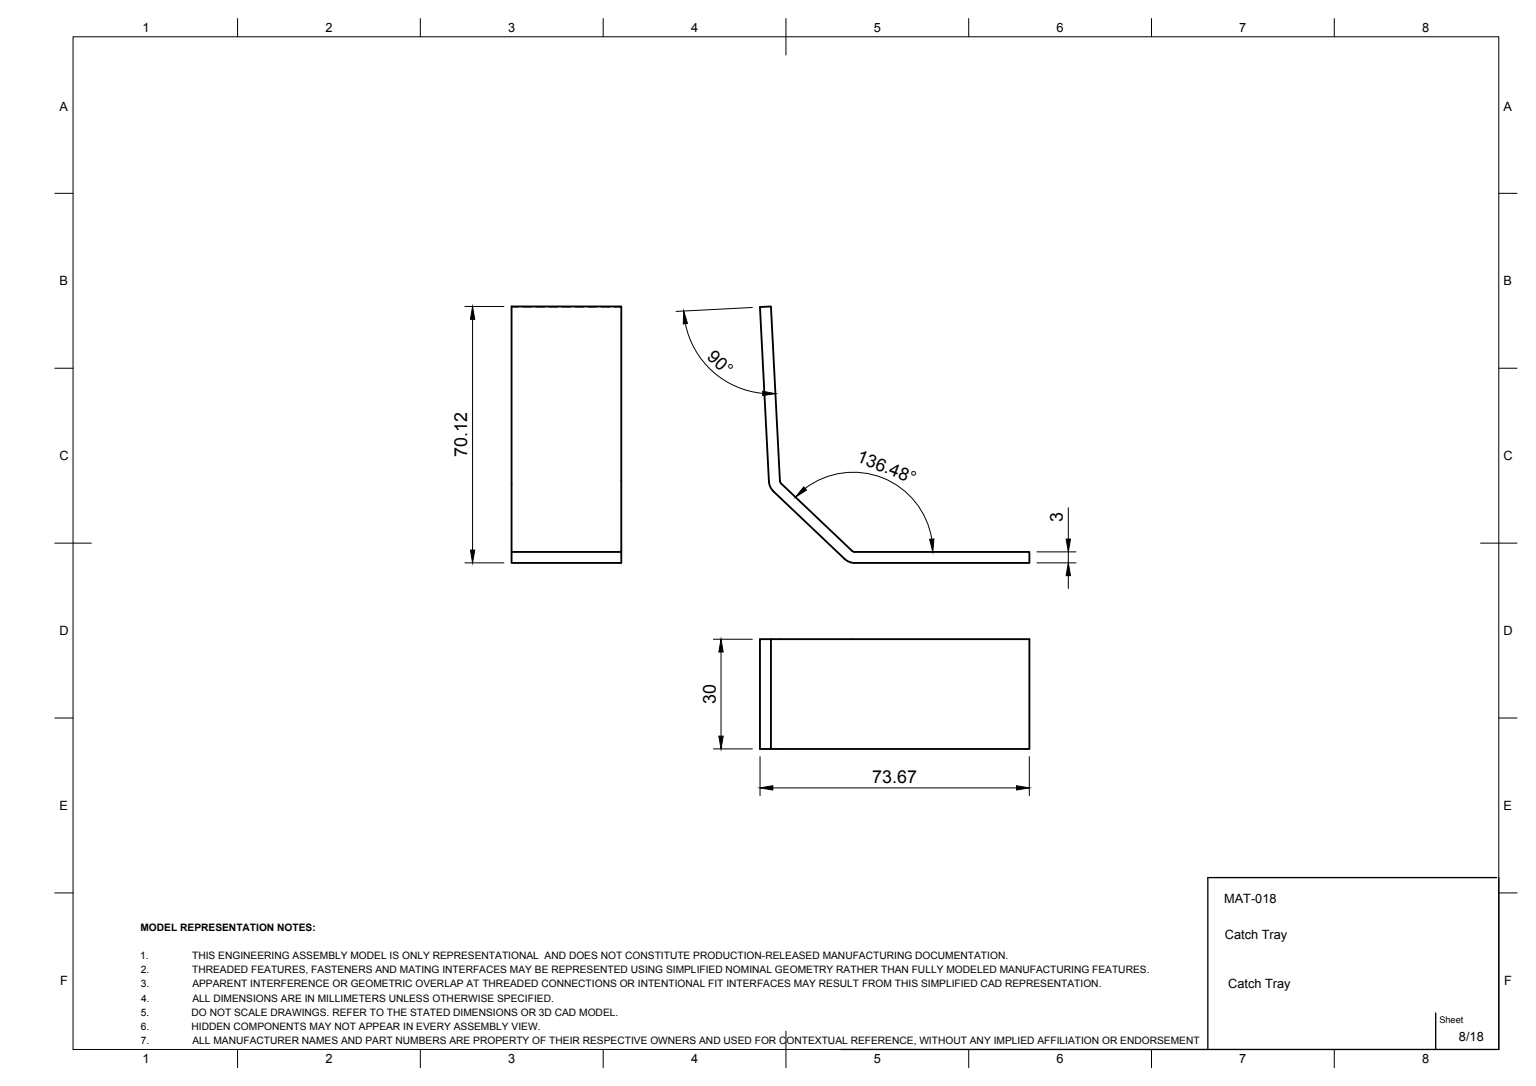
ISO-10303-21;
HEADER;
/* Generated by software containing ST-Developer
 * from STEP Tools, Inc. (www.steptools.com) 
 */

FILE_DESCRIPTION(
/* description */ ('STEP AP214'),
/* implementation_level */ '2;1');

FILE_NAME(
/* name */ 'Catch Tray.step',
/* time_stamp */ '2026-11-14T06:16:09-08:00',
/* author */ (''),
/* organization */ (''),
/* preprocessor_version */ 'ST-DEVELOPER v20.2',
/* originating_system */ 'Autodesk Translation Framework v15.17.0.0',
/* authorisation */ '');

FILE_SCHEMA (('AUTOMOTIVE_DESIGN { 1 0 10303 214 3 1 1 }'));
ENDSEC;

DATA;
#10=MECHANICAL_DESIGN_GEOMETRIC_PRESENTATION_REPRESENTATION('',(#352),#18006);
#320=SHAPE_REPRESENTATION_RELATIONSHIP('SRR','None',#18076,#336);
#336=ADVANCED_BREP_SHAPE_REPRESENTATION('',(#368),#17993);
#352=STYLED_ITEM('',(#18170),#368);
#368=MANIFOLD_SOLID_BREP('Body1',#9561);
#692=PLANE('',#10212);
#693=PLANE('',#10215);
#694=PLANE('',#10216);
#695=PLANE('',#10219);
#696=PLANE('',#10220);
#697=PLANE('',#10223);
#698=PLANE('',#10224);
#699=PLANE('',#10227);
#700=PLANE('',#10228);
#701=PLANE('',#10229);
#702=PLANE('',#10230);
#703=PLANE('',#10232);
#704=PLANE('',#10234);
#705=PLANE('',#10235);
#706=PLANE('',#10236);
#707=PLANE('',#10238);
#708=PLANE('',#10240);
#709=PLANE('',#10241);
#1117=FACE_OUTER_BOUND('',#1769,.T.);
#1118=FACE_OUTER_BOUND('',#1770,.T.);
#1119=FACE_OUTER_BOUND('',#1771,.T.);
#1120=FACE_OUTER_BOUND('',#1772,.T.);
#1121=FACE_OUTER_BOUND('',#1773,.T.);
#1122=FACE_OUTER_BOUND('',#1774,.T.);
#1123=FACE_OUTER_BOUND('',#1775,.T.);
#1124=FACE_OUTER_BOUND('',#1776,.T.);
#1125=FACE_OUTER_BOUND('',#1777,.T.);
#1126=FACE_OUTER_BOUND('',#1778,.T.);
#1127=FACE_OUTER_BOUND('',#1779,.T.);
#1128=FACE_OUTER_BOUND('',#1780,.T.);
#1129=FACE_OUTER_BOUND('',#1781,.T.);
#1130=FACE_OUTER_BOUND('',#1782,.T.);
#1131=FACE_OUTER_BOUND('',#1783,.T.);
#1132=FACE_OUTER_BOUND('',#1784,.T.);
#1133=FACE_OUTER_BOUND('',#1785,.T.);
#1134=FACE_OUTER_BOUND('',#1786,.T.);
#1135=FACE_OUTER_BOUND('',#1787,.T.);
#1136=FACE_OUTER_BOUND('',#1788,.T.);
#1137=FACE_OUTER_BOUND('',#1789,.T.);
#1138=FACE_OUTER_BOUND('',#1790,.T.);
#1769=EDGE_LOOP('',(#7428,#7429,#7430,#7431));
#1770=EDGE_LOOP('',(#7432,#7433,#7434,#7435));
#1771=EDGE_LOOP('',(#7436,#7437,#7438,#7439));
#1772=EDGE_LOOP('',(#7440,#7441,#7442,#7443));
#1773=EDGE_LOOP('',(#7444,#7445,#7446,#7447));
#1774=EDGE_LOOP('',(#7448,#7449,#7450,#7451));
#1775=EDGE_LOOP('',(#7452,#7453,#7454,#7455));
#1776=EDGE_LOOP('',(#7456,#7457,#7458,#7459));
#1777=EDGE_LOOP('',(#7460,#7461,#7462,#7463));
#1778=EDGE_LOOP('',(#7464,#7465,#7466,#7467));
#1779=EDGE_LOOP('',(#7468,#7469,#7470,#7471));
#1780=EDGE_LOOP('',(#7472,#7473,#7474,#7475));
#1781=EDGE_LOOP('',(#7476,#7477,#7478,#7479));
#1782=EDGE_LOOP('',(#7480,#7481,#7482,#7483));
#1783=EDGE_LOOP('',(#7484,#7485,#7486,#7487));
#1784=EDGE_LOOP('',(#7488,#7489,#7490,#7491));
#1785=EDGE_LOOP('',(#7492,#7493,#7494,#7495));
#1786=EDGE_LOOP('',(#7496,#7497,#7498,#7499));
#1787=EDGE_LOOP('',(#7500,#7501,#7502,#7503));
#1788=EDGE_LOOP('',(#7504,#7505,#7506,#7507));
#1789=EDGE_LOOP('',(#7508,#7509,#7510,#7511));
#1790=EDGE_LOOP('',(#7512,#7513,#7514,#7515));
#2574=LINE('',#15105,#3298);
#2575=LINE('',#15109,#3299);
#2576=LINE('',#15113,#3300);
#2577=LINE('',#15115,#3301);
#2578=LINE('',#15116,#3302);
#2579=LINE('',#15120,#3303);
#2580=LINE('',#15124,#3304);
#2581=LINE('',#15128,#3305);
#2582=LINE('',#15130,#3306);
#2583=LINE('',#15131,#3307);
#2584=LINE('',#15135,#3308);
#2585=LINE('',#15140,#3309);
#2586=LINE('',#15142,#3310);
#2587=LINE('',#15143,#3311);
#2588=LINE('',#15147,#3312);
#2589=LINE('',#15151,#3313);
#2590=LINE('',#15154,#3314);
#2591=LINE('',#15155,#3315);
#2592=LINE('',#15158,#3316);
#2593=LINE('',#15159,#3317);
#2594=LINE('',#15160,#3318);
#2595=LINE('',#15163,#3319);
#2596=LINE('',#15164,#3320);
#2597=LINE('',#15166,#3321);
#2598=LINE('',#15167,#3322);
#2599=LINE('',#15169,#3323);
#2600=LINE('',#15171,#3324);
#2601=LINE('',#15173,#3325);
#2602=LINE('',#15176,#3326);
#2603=LINE('',#15177,#3327);
#2604=LINE('',#15180,#3328);
#2605=LINE('',#15181,#3329);
#2606=LINE('',#15183,#3330);
#2607=LINE('',#15184,#3331);
#2608=LINE('',#15186,#3332);
#2609=LINE('',#15188,#3333);
#3298=VECTOR('',#12247,1000.);
#3299=VECTOR('',#12250,1000.);
#3300=VECTOR('',#12255,1000.);
#3301=VECTOR('',#12256,1000.);
#3302=VECTOR('',#12257,1000.);
#3303=VECTOR('',#12260,1000.);
#3304=VECTOR('',#12263,1000.);
#3305=VECTOR('',#12268,1000.);
#3306=VECTOR('',#12269,1000.);
#3307=VECTOR('',#12270,1000.);
#3308=VECTOR('',#12273,1000.);
#3309=VECTOR('',#12280,1000.);
#3310=VECTOR('',#12281,1000.);
#3311=VECTOR('',#12282,1000.);
#3312=VECTOR('',#12285,1000.);
#3313=VECTOR('',#12288,1000.);
#3314=VECTOR('',#12293,1000.);
#3315=VECTOR('',#12294,1000.);
#3316=VECTOR('',#12297,1000.);
#3317=VECTOR('',#12298,1000.);
#3318=VECTOR('',#12299,1000.);
#3319=VECTOR('',#12302,1000.);
#3320=VECTOR('',#12303,1000.);
#3321=VECTOR('',#12306,1000.);
#3322=VECTOR('',#12307,1000.);
#3323=VECTOR('',#12310,1000.);
#3324=VECTOR('',#12313,1000.);
#3325=VECTOR('',#12316,1000.);
#3326=VECTOR('',#12319,1000.);
#3327=VECTOR('',#12320,1000.);
#3328=VECTOR('',#12323,1000.);
#3329=VECTOR('',#12324,1000.);
#3330=VECTOR('',#12327,1000.);
#3331=VECTOR('',#12328,1000.);
#3332=VECTOR('',#12331,1000.);
#3333=VECTOR('',#12334,1000.);
#3736=CIRCLE('',#10213,4.);
#3737=CIRCLE('',#10214,1.);
#3738=CIRCLE('',#10217,4.);
#3739=CIRCLE('',#10218,1.);
#3740=CIRCLE('',#10221,4.);
#3741=CIRCLE('',#10222,1.);
#3742=CIRCLE('',#10225,4.);
#3743=CIRCLE('',#10226,1.);
#4385=VERTEX_POINT('',#15103);
#4386=VERTEX_POINT('',#15104);
#4387=VERTEX_POINT('',#15106);
#4388=VERTEX_POINT('',#15108);
#4389=VERTEX_POINT('',#15112);
#4390=VERTEX_POINT('',#15114);
#4391=VERTEX_POINT('',#15118);
#4392=VERTEX_POINT('',#15119);
#4393=VERTEX_POINT('',#15121);
#4394=VERTEX_POINT('',#15123);
#4395=VERTEX_POINT('',#15127);
#4396=VERTEX_POINT('',#15129);
#4397=VERTEX_POINT('',#15133);
#4398=VERTEX_POINT('',#15134);
#4399=VERTEX_POINT('',#15139);
#4400=VERTEX_POINT('',#15141);
#4401=VERTEX_POINT('',#15145);
#4402=VERTEX_POINT('',#15146);
#4403=VERTEX_POINT('',#15148);
#4404=VERTEX_POINT('',#15150);
#4405=VERTEX_POINT('',#15157);
#4406=VERTEX_POINT('',#15162);
#4407=VERTEX_POINT('',#15175);
#4408=VERTEX_POINT('',#15179);
#5462=EDGE_CURVE('',#4385,#4386,#2574,.T.);
#5463=EDGE_CURVE('',#4387,#4385,#3736,.T.);
#5464=EDGE_CURVE('',#4388,#4387,#2575,.T.);
#5465=EDGE_CURVE('',#4388,#4386,#3737,.T.);
#5466=EDGE_CURVE('',#4385,#4389,#2576,.T.);
#5467=EDGE_CURVE('',#4386,#4390,#2577,.T.);
#5468=EDGE_CURVE('',#4390,#4389,#2578,.T.);
#5469=EDGE_CURVE('',#4391,#4392,#2579,.T.);
#5470=EDGE_CURVE('',#4391,#4393,#3738,.T.);
#5471=EDGE_CURVE('',#4394,#4393,#2580,.T.);
#5472=EDGE_CURVE('',#4392,#4394,#3739,.T.);
#5473=EDGE_CURVE('',#4395,#4391,#2581,.T.);
#5474=EDGE_CURVE('',#4396,#4392,#2582,.T.);
#5475=EDGE_CURVE('',#4396,#4395,#2583,.T.);
#5476=EDGE_CURVE('',#4397,#4398,#2584,.T.);
#5477=EDGE_CURVE('',#4389,#4397,#3740,.T.);
#5478=EDGE_CURVE('',#4390,#4398,#3741,.T.);
#5479=EDGE_CURVE('',#4397,#4399,#2585,.T.);
#5480=EDGE_CURVE('',#4398,#4400,#2586,.T.);
#5481=EDGE_CURVE('',#4399,#4400,#2587,.T.);
#5482=EDGE_CURVE('',#4401,#4402,#2588,.T.);
#5483=EDGE_CURVE('',#4401,#4403,#3742,.T.);
#5484=EDGE_CURVE('',#4404,#4403,#2589,.T.);
#5485=EDGE_CURVE('',#4402,#4404,#3743,.T.);
#5486=EDGE_CURVE('',#4393,#4401,#2590,.T.);
#5487=EDGE_CURVE('',#4394,#4402,#2591,.T.);
#5488=EDGE_CURVE('',#4404,#4405,#2592,.T.);
#5489=EDGE_CURVE('',#4400,#4405,#2593,.T.);
#5490=EDGE_CURVE('',#4398,#4404,#2594,.T.);
#5491=EDGE_CURVE('',#4406,#4405,#2595,.T.);
#5492=EDGE_CURVE('',#4399,#4406,#2596,.T.);
#5493=EDGE_CURVE('',#4403,#4406,#2597,.T.);
#5494=EDGE_CURVE('',#4397,#4403,#2598,.T.);
#5495=EDGE_CURVE('',#4389,#4401,#2599,.T.);
#5496=EDGE_CURVE('',#4385,#4393,#2600,.T.);
#5497=EDGE_CURVE('',#4387,#4391,#2601,.T.);
#5498=EDGE_CURVE('',#4407,#4395,#2602,.T.);
#5499=EDGE_CURVE('',#4407,#4387,#2603,.T.);
#5500=EDGE_CURVE('',#4408,#4396,#2604,.T.);
#5501=EDGE_CURVE('',#4408,#4407,#2605,.T.);
#5502=EDGE_CURVE('',#4388,#4392,#2606,.T.);
#5503=EDGE_CURVE('',#4408,#4388,#2607,.T.);
#5504=EDGE_CURVE('',#4386,#4394,#2608,.T.);
#5505=EDGE_CURVE('',#4390,#4402,#2609,.T.);
#7428=ORIENTED_EDGE('',*,*,#5462,.F.);
#7429=ORIENTED_EDGE('',*,*,#5463,.F.);
#7430=ORIENTED_EDGE('',*,*,#5464,.F.);
#7431=ORIENTED_EDGE('',*,*,#5465,.T.);
#7432=ORIENTED_EDGE('',*,*,#5466,.F.);
#7433=ORIENTED_EDGE('',*,*,#5462,.T.);
#7434=ORIENTED_EDGE('',*,*,#5467,.T.);
#7435=ORIENTED_EDGE('',*,*,#5468,.T.);
#7436=ORIENTED_EDGE('',*,*,#5469,.F.);
#7437=ORIENTED_EDGE('',*,*,#5470,.T.);
#7438=ORIENTED_EDGE('',*,*,#5471,.F.);
#7439=ORIENTED_EDGE('',*,*,#5472,.F.);
#7440=ORIENTED_EDGE('',*,*,#5473,.T.);
#7441=ORIENTED_EDGE('',*,*,#5469,.T.);
#7442=ORIENTED_EDGE('',*,*,#5474,.F.);
#7443=ORIENTED_EDGE('',*,*,#5475,.T.);
#7444=ORIENTED_EDGE('',*,*,#5476,.F.);
#7445=ORIENTED_EDGE('',*,*,#5477,.F.);
#7446=ORIENTED_EDGE('',*,*,#5468,.F.);
#7447=ORIENTED_EDGE('',*,*,#5478,.T.);
#7448=ORIENTED_EDGE('',*,*,#5479,.F.);
#7449=ORIENTED_EDGE('',*,*,#5476,.T.);
#7450=ORIENTED_EDGE('',*,*,#5480,.T.);
#7451=ORIENTED_EDGE('',*,*,#5481,.F.);
#7452=ORIENTED_EDGE('',*,*,#5482,.F.);
#7453=ORIENTED_EDGE('',*,*,#5483,.T.);
#7454=ORIENTED_EDGE('',*,*,#5484,.F.);
#7455=ORIENTED_EDGE('',*,*,#5485,.F.);
#7456=ORIENTED_EDGE('',*,*,#5486,.T.);
#7457=ORIENTED_EDGE('',*,*,#5482,.T.);
#7458=ORIENTED_EDGE('',*,*,#5487,.F.);
#7459=ORIENTED_EDGE('',*,*,#5471,.T.);
#7460=ORIENTED_EDGE('',*,*,#5488,.T.);
#7461=ORIENTED_EDGE('',*,*,#5489,.F.);
#7462=ORIENTED_EDGE('',*,*,#5480,.F.);
#7463=ORIENTED_EDGE('',*,*,#5490,.T.);
#7464=ORIENTED_EDGE('',*,*,#5491,.F.);
#7465=ORIENTED_EDGE('',*,*,#5492,.F.);
#7466=ORIENTED_EDGE('',*,*,#5481,.T.);
#7467=ORIENTED_EDGE('',*,*,#5489,.T.);
#7468=ORIENTED_EDGE('',*,*,#5493,.F.);
#7469=ORIENTED_EDGE('',*,*,#5494,.F.);
#7470=ORIENTED_EDGE('',*,*,#5479,.T.);
#7471=ORIENTED_EDGE('',*,*,#5492,.T.);
#7472=ORIENTED_EDGE('',*,*,#5483,.F.);
#7473=ORIENTED_EDGE('',*,*,#5495,.F.);
#7474=ORIENTED_EDGE('',*,*,#5477,.T.);
#7475=ORIENTED_EDGE('',*,*,#5494,.T.);
#7476=ORIENTED_EDGE('',*,*,#5486,.F.);
#7477=ORIENTED_EDGE('',*,*,#5496,.F.);
#7478=ORIENTED_EDGE('',*,*,#5466,.T.);
#7479=ORIENTED_EDGE('',*,*,#5495,.T.);
#7480=ORIENTED_EDGE('',*,*,#5470,.F.);
#7481=ORIENTED_EDGE('',*,*,#5497,.F.);
#7482=ORIENTED_EDGE('',*,*,#5463,.T.);
#7483=ORIENTED_EDGE('',*,*,#5496,.T.);
#7484=ORIENTED_EDGE('',*,*,#5473,.F.);
#7485=ORIENTED_EDGE('',*,*,#5498,.F.);
#7486=ORIENTED_EDGE('',*,*,#5499,.T.);
#7487=ORIENTED_EDGE('',*,*,#5497,.T.);
#7488=ORIENTED_EDGE('',*,*,#5475,.F.);
#7489=ORIENTED_EDGE('',*,*,#5500,.F.);
#7490=ORIENTED_EDGE('',*,*,#5501,.T.);
#7491=ORIENTED_EDGE('',*,*,#5498,.T.);
#7492=ORIENTED_EDGE('',*,*,#5474,.T.);
#7493=ORIENTED_EDGE('',*,*,#5502,.F.);
#7494=ORIENTED_EDGE('',*,*,#5503,.F.);
#7495=ORIENTED_EDGE('',*,*,#5500,.T.);
#7496=ORIENTED_EDGE('',*,*,#5472,.T.);
#7497=ORIENTED_EDGE('',*,*,#5504,.F.);
#7498=ORIENTED_EDGE('',*,*,#5465,.F.);
#7499=ORIENTED_EDGE('',*,*,#5502,.T.);
#7500=ORIENTED_EDGE('',*,*,#5487,.T.);
#7501=ORIENTED_EDGE('',*,*,#5505,.F.);
#7502=ORIENTED_EDGE('',*,*,#5467,.F.);
#7503=ORIENTED_EDGE('',*,*,#5504,.T.);
#7504=ORIENTED_EDGE('',*,*,#5485,.T.);
#7505=ORIENTED_EDGE('',*,*,#5490,.F.);
#7506=ORIENTED_EDGE('',*,*,#5478,.F.);
#7507=ORIENTED_EDGE('',*,*,#5505,.T.);
#7508=ORIENTED_EDGE('',*,*,#5503,.T.);
#7509=ORIENTED_EDGE('',*,*,#5464,.T.);
#7510=ORIENTED_EDGE('',*,*,#5499,.F.);
#7511=ORIENTED_EDGE('',*,*,#5501,.F.);
#7512=ORIENTED_EDGE('',*,*,#5488,.F.);
#7513=ORIENTED_EDGE('',*,*,#5484,.T.);
#7514=ORIENTED_EDGE('',*,*,#5493,.T.);
#7515=ORIENTED_EDGE('',*,*,#5491,.T.);
#8894=CYLINDRICAL_SURFACE('',#10231,4.);
#8895=CYLINDRICAL_SURFACE('',#10233,4.);
#8896=CYLINDRICAL_SURFACE('',#10237,1.);
#8897=CYLINDRICAL_SURFACE('',#10239,1.);
#9256=ADVANCED_FACE('',(#1117),#692,.T.);
#9257=ADVANCED_FACE('',(#1118),#693,.T.);
#9258=ADVANCED_FACE('',(#1119),#694,.T.);
#9259=ADVANCED_FACE('',(#1120),#695,.T.);
#9260=ADVANCED_FACE('',(#1121),#696,.T.);
#9261=ADVANCED_FACE('',(#1122),#697,.T.);
#9262=ADVANCED_FACE('',(#1123),#698,.T.);
#9263=ADVANCED_FACE('',(#1124),#699,.T.);
#9264=ADVANCED_FACE('',(#1125),#700,.F.);
#9265=ADVANCED_FACE('',(#1126),#701,.T.);
#9266=ADVANCED_FACE('',(#1127),#702,.T.);
#9267=ADVANCED_FACE('',(#1128),#8894,.T.);
#9268=ADVANCED_FACE('',(#1129),#703,.T.);
#9269=ADVANCED_FACE('',(#1130),#8895,.T.);
#9270=ADVANCED_FACE('',(#1131),#704,.T.);
#9271=ADVANCED_FACE('',(#1132),#705,.T.);
#9272=ADVANCED_FACE('',(#1133),#706,.F.);
#9273=ADVANCED_FACE('',(#1134),#8896,.F.);
#9274=ADVANCED_FACE('',(#1135),#707,.F.);
#9275=ADVANCED_FACE('',(#1136),#8897,.F.);
#9276=ADVANCED_FACE('',(#1137),#708,.T.);
#9277=ADVANCED_FACE('',(#1138),#709,.F.);
#9561=CLOSED_SHELL('',(#9256,#9257,#9258,#9259,#9260,#9261,#9262,#9263,
#9264,#9265,#9266,#9267,#9268,#9269,#9270,#9271,#9272,#9273,#9274,#9275,
#9276,#9277));
#10211=AXIS2_PLACEMENT_3D('',#15101,#12243,#12244);
#10212=AXIS2_PLACEMENT_3D('',#15102,#12245,#12246);
#10213=AXIS2_PLACEMENT_3D('',#15107,#12248,#12249);
#10214=AXIS2_PLACEMENT_3D('',#15110,#12251,#12252);
#10215=AXIS2_PLACEMENT_3D('',#15111,#12253,#12254);
#10216=AXIS2_PLACEMENT_3D('',#15117,#12258,#12259);
#10217=AXIS2_PLACEMENT_3D('',#15122,#12261,#12262);
#10218=AXIS2_PLACEMENT_3D('',#15125,#12264,#12265);
#10219=AXIS2_PLACEMENT_3D('',#15126,#12266,#12267);
#10220=AXIS2_PLACEMENT_3D('',#15132,#12271,#12272);
#10221=AXIS2_PLACEMENT_3D('',#15136,#12274,#12275);
#10222=AXIS2_PLACEMENT_3D('',#15137,#12276,#12277);
#10223=AXIS2_PLACEMENT_3D('',#15138,#12278,#12279);
#10224=AXIS2_PLACEMENT_3D('',#15144,#12283,#12284);
#10225=AXIS2_PLACEMENT_3D('',#15149,#12286,#12287);
#10226=AXIS2_PLACEMENT_3D('',#15152,#12289,#12290);
#10227=AXIS2_PLACEMENT_3D('',#15153,#12291,#12292);
#10228=AXIS2_PLACEMENT_3D('',#15156,#12295,#12296);
#10229=AXIS2_PLACEMENT_3D('',#15161,#12300,#12301);
#10230=AXIS2_PLACEMENT_3D('',#15165,#12304,#12305);
#10231=AXIS2_PLACEMENT_3D('',#15168,#12308,#12309);
#10232=AXIS2_PLACEMENT_3D('',#15170,#12311,#12312);
#10233=AXIS2_PLACEMENT_3D('',#15172,#12314,#12315);
#10234=AXIS2_PLACEMENT_3D('',#15174,#12317,#12318);
#10235=AXIS2_PLACEMENT_3D('',#15178,#12321,#12322);
#10236=AXIS2_PLACEMENT_3D('',#15182,#12325,#12326);
#10237=AXIS2_PLACEMENT_3D('',#15185,#12329,#12330);
#10238=AXIS2_PLACEMENT_3D('',#15187,#12332,#12333);
#10239=AXIS2_PLACEMENT_3D('',#15189,#12335,#12336);
#10240=AXIS2_PLACEMENT_3D('',#15190,#12337,#12338);
#10241=AXIS2_PLACEMENT_3D('',#15191,#12339,#12340);
#12243=DIRECTION('axis',(0.,0.,1.));
#12244=DIRECTION('refdir',(1.,0.,0.));
#12245=DIRECTION('center_axis',(0.,0.,1.));
#12246=DIRECTION('ref_axis',(1.,0.,0.));
#12247=DIRECTION('',(0.,-1.,0.));
#12248=DIRECTION('center_axis',(0.,0.,-1.));
#12249=DIRECTION('ref_axis',(1.,0.,0.));
#12250=DIRECTION('',(-0.688642993486688,0.72510056373009,0.));
#12251=DIRECTION('center_axis',(0.,0.,-1.));
#12252=DIRECTION('ref_axis',(1.,0.,0.));
#12253=DIRECTION('center_axis',(0.,0.,1.));
#12254=DIRECTION('ref_axis',(1.,0.,0.));
#12255=DIRECTION('',(1.,0.,0.));
#12256=DIRECTION('',(1.,0.,0.));
#12257=DIRECTION('',(0.,1.,0.));
#12258=DIRECTION('center_axis',(0.,0.,-1.));
#12259=DIRECTION('ref_axis',(-1.,0.,0.));
#12260=DIRECTION('',(0.688642993486688,-0.72510056373009,0.));
#12261=DIRECTION('center_axis',(0.,0.,-1.));
#12262=DIRECTION('ref_axis',(1.,0.,0.));
#12263=DIRECTION('',(0.,1.,0.));
#12264=DIRECTION('center_axis',(0.,0.,-1.));
#12265=DIRECTION('ref_axis',(1.,0.,0.));
#12266=DIRECTION('center_axis',(0.,0.,-1.));
#12267=DIRECTION('ref_axis',(-1.,0.,0.));
#12268=DIRECTION('',(0.725100563730095,0.688642993486682,0.));
#12269=DIRECTION('',(0.725100563730095,0.688642993486682,0.));
#12270=DIRECTION('',(-0.688642993486682,0.725100563730095,0.));
#12271=DIRECTION('center_axis',(0.,0.,1.));
#12272=DIRECTION('ref_axis',(1.,0.,0.));
#12273=DIRECTION('',(-0.688642993486681,-0.725100563730095,0.));
#12274=DIRECTION('center_axis',(0.,0.,-1.));
#12275=DIRECTION('ref_axis',(1.,-1.73472347597681E-15,0.));
#12276=DIRECTION('center_axis',(0.,0.,-1.));
#12277=DIRECTION('ref_axis',(1.,0.,0.));
#12278=DIRECTION('center_axis',(0.,0.,1.));
#12279=DIRECTION('ref_axis',(1.,0.,0.));
#12280=DIRECTION('',(0.725100563730095,-0.688642993486682,0.));
#12281=DIRECTION('',(0.725100563730095,-0.688642993486682,0.));
#12282=DIRECTION('',(-0.688642993486681,-0.725100563730095,0.));
#12283=DIRECTION('center_axis',(0.,0.,-1.));
#12284=DIRECTION('ref_axis',(-1.,0.,0.));
#12285=DIRECTION('',(0.,-1.,0.));
#12286=DIRECTION('center_axis',(0.,0.,-1.));
#12287=DIRECTION('ref_axis',(1.,-1.73472347597681E-15,0.));
#12288=DIRECTION('',(0.688642993486681,0.725100563730095,0.));
#12289=DIRECTION('center_axis',(0.,0.,-1.));
#12290=DIRECTION('ref_axis',(1.,0.,0.));
#12291=DIRECTION('center_axis',(0.,0.,-1.));
#12292=DIRECTION('ref_axis',(-1.,0.,0.));
#12293=DIRECTION('',(1.,0.,0.));
#12294=DIRECTION('',(1.,0.,0.));
#12295=DIRECTION('center_axis',(0.688642993486682,0.725100563730095,0.));
#12296=DIRECTION('ref_axis',(-0.725100563730095,0.688642993486682,0.));
#12297=DIRECTION('',(0.725100563730095,-0.688642993486682,0.));
#12298=DIRECTION('',(0.,0.,-1.));
#12299=DIRECTION('',(0.,0.,-1.));
#12300=DIRECTION('center_axis',(0.725100563730096,-0.688642993486682,0.));
#12301=DIRECTION('ref_axis',(0.688642993486682,0.725100563730096,0.));
#12302=DIRECTION('',(-0.688642993486681,-0.725100563730095,0.));
#12303=DIRECTION('',(0.,0.,-1.));
#12304=DIRECTION('center_axis',(0.688642993486682,0.725100563730095,0.));
#12305=DIRECTION('ref_axis',(-0.725100563730095,0.688642993486682,0.));
#12306=DIRECTION('',(0.725100563730095,-0.688642993486682,0.));
#12307=DIRECTION('',(0.,0.,-1.));
#12308=DIRECTION('center_axis',(0.,0.,-1.));
#12309=DIRECTION('ref_axis',(-1.,0.,0.));
#12310=DIRECTION('',(0.,0.,-1.));
#12311=DIRECTION('center_axis',(0.,1.,0.));
#12312=DIRECTION('ref_axis',(0.,0.,1.));
#12313=DIRECTION('',(0.,0.,-1.));
#12314=DIRECTION('center_axis',(0.,0.,-1.));
#12315=DIRECTION('ref_axis',(-1.,0.,0.));
#12316=DIRECTION('',(0.,0.,-1.));
#12317=DIRECTION('center_axis',(-0.688642993486682,0.725100563730095,0.));
#12318=DIRECTION('ref_axis',(-0.725100563730095,-0.688642993486682,0.));
#12319=DIRECTION('',(0.,0.,-1.));
#12320=DIRECTION('',(0.725100563730095,0.688642993486682,0.));
#12321=DIRECTION('center_axis',(-0.725100563730095,-0.688642993486682,0.));
#12322=DIRECTION('ref_axis',(0.688642993486682,-0.725100563730095,0.));
#12323=DIRECTION('',(0.,0.,-1.));
#12324=DIRECTION('',(-0.688642993486682,0.725100563730095,0.));
#12325=DIRECTION('center_axis',(-0.688642993486682,0.725100563730095,0.));
#12326=DIRECTION('ref_axis',(-0.725100563730095,-0.688642993486682,0.));
#12327=DIRECTION('',(0.,0.,-1.));
#12328=DIRECTION('',(0.725100563730095,0.688642993486682,0.));
#12329=DIRECTION('center_axis',(0.,0.,-1.));
#12330=DIRECTION('ref_axis',(-1.,0.,0.));
#12331=DIRECTION('',(0.,0.,-1.));
#12332=DIRECTION('center_axis',(0.,1.,0.));
#12333=DIRECTION('ref_axis',(0.,0.,1.));
#12334=DIRECTION('',(0.,0.,-1.));
#12335=DIRECTION('center_axis',(0.,0.,-1.));
#12336=DIRECTION('ref_axis',(-1.,0.,0.));
#12337=DIRECTION('center_axis',(0.,0.,1.));
#12338=DIRECTION('ref_axis',(1.,0.,0.));
#12339=DIRECTION('center_axis',(0.,0.,1.));
#12340=DIRECTION('ref_axis',(1.,0.,0.));
#15101=CARTESIAN_POINT('',(0.,0.,0.));
#15102=CARTESIAN_POINT('Origin',(37.3967602305982,34.,30.));
#15103=CARTESIAN_POINT('',(37.3967602305982,34.,30.));
#15104=CARTESIAN_POINT('',(37.3967602305982,31.,30.));
#15105=CARTESIAN_POINT('',(37.3967602305982,34.,30.));
#15106=CARTESIAN_POINT('',(34.6421882566514,32.9004022549204,30.));
#15107=CARTESIAN_POINT('Origin',(37.3967602305982,30.,30.));
#15108=CARTESIAN_POINT('',(36.7081172371115,30.7251005637301,30.));
#15109=CARTESIAN_POINT('',(36.7081172371115,30.7251005637301,30.));
#15110=CARTESIAN_POINT('Origin',(37.3967602305982,30.,30.));
#15111=CARTESIAN_POINT('Origin',(36.7081172371115,30.7251005637301,30.));
#15112=CARTESIAN_POINT('',(64.2032397694018,34.,30.));
#15113=CARTESIAN_POINT('',(35.8,34.,30.));
#15114=CARTESIAN_POINT('',(64.2032397694018,31.,30.));
#15115=CARTESIAN_POINT('',(35.8,31.,30.));
#15116=CARTESIAN_POINT('',(64.2032397694018,31.,30.));
#15117=CARTESIAN_POINT('Origin',(34.6421882566514,32.9004022549204,0.));
#15118=CARTESIAN_POINT('',(34.6421882566514,32.9004022549204,0.));
#15119=CARTESIAN_POINT('',(36.7081172371115,30.7251005637301,0.));
#15120=CARTESIAN_POINT('',(34.6421882566514,32.9004022549204,0.));
#15121=CARTESIAN_POINT('',(37.3967602305982,34.,0.));
#15122=CARTESIAN_POINT('Origin',(37.3967602305982,30.,0.));
#15123=CARTESIAN_POINT('',(37.3967602305982,31.,0.));
#15124=CARTESIAN_POINT('',(37.3967602305982,31.,0.));
#15125=CARTESIAN_POINT('Origin',(37.3967602305982,30.,0.));
#15126=CARTESIAN_POINT('Origin',(37.3967602305982,31.,0.));
#15127=CARTESIAN_POINT('',(0.,0.,0.));
#15128=CARTESIAN_POINT('',(0.,0.,0.));
#15129=CARTESIAN_POINT('',(2.06592898046005,-2.17530169119028,0.));
#15130=CARTESIAN_POINT('',(2.06592898046005,-2.17530169119028,0.));
#15131=CARTESIAN_POINT('',(2.06592898046005,-2.17530169119028,0.));
#15132=CARTESIAN_POINT('Origin',(66.9578117433485,32.9004022549204,30.));
#15133=CARTESIAN_POINT('',(66.9578117433485,32.9004022549204,30.));
#15134=CARTESIAN_POINT('',(64.8918827628885,30.7251005637301,30.));
#15135=CARTESIAN_POINT('',(66.9578117433485,32.9004022549204,30.));
#15136=CARTESIAN_POINT('Origin',(64.2032397694018,30.,30.));
#15137=CARTESIAN_POINT('Origin',(64.2032397694018,30.,30.));
#15138=CARTESIAN_POINT('Origin',(64.2032397694018,31.,30.));
#15139=CARTESIAN_POINT('',(101.6,0.,30.));
#15140=CARTESIAN_POINT('',(65.8,34.,30.));
#15141=CARTESIAN_POINT('',(99.53407101954,-2.17530169119028,30.));
#15142=CARTESIAN_POINT('',(63.73407101954,31.8246983088097,30.));
#15143=CARTESIAN_POINT('',(101.6,0.,30.));
#15144=CARTESIAN_POINT('Origin',(64.2032397694018,34.,0.));
#15145=CARTESIAN_POINT('',(64.2032397694018,34.,0.));
#15146=CARTESIAN_POINT('',(64.2032397694018,31.,0.));
#15147=CARTESIAN_POINT('',(64.2032397694018,34.,0.));
#15148=CARTESIAN_POINT('',(66.9578117433485,32.9004022549204,0.));
#15149=CARTESIAN_POINT('Origin',(64.2032397694018,30.,0.));
#15150=CARTESIAN_POINT('',(64.8918827628885,30.7251005637301,0.));
#15151=CARTESIAN_POINT('',(64.8918827628885,30.7251005637301,0.));
#15152=CARTESIAN_POINT('Origin',(64.2032397694018,30.,0.));
#15153=CARTESIAN_POINT('Origin',(64.8918827628885,30.7251005637301,0.));
#15154=CARTESIAN_POINT('',(35.8,34.,0.));
#15155=CARTESIAN_POINT('',(35.8,31.,0.));
#15156=CARTESIAN_POINT('Origin',(63.73407101954,31.8246983088097,30.));
#15157=CARTESIAN_POINT('',(99.53407101954,-2.17530169119028,0.));
#15158=CARTESIAN_POINT('',(63.73407101954,31.8246983088097,0.));
#15159=CARTESIAN_POINT('',(99.53407101954,-2.17530169119028,30.));
#15160=CARTESIAN_POINT('',(64.8918827628885,30.7251005637301,30.));
#15161=CARTESIAN_POINT('Origin',(101.6,0.,30.));
#15162=CARTESIAN_POINT('',(101.6,0.,0.));
#15163=CARTESIAN_POINT('',(101.6,0.,0.));
#15164=CARTESIAN_POINT('',(101.6,0.,30.));
#15165=CARTESIAN_POINT('Origin',(65.8,34.,30.));
#15166=CARTESIAN_POINT('',(65.8,34.,0.));
#15167=CARTESIAN_POINT('',(66.9578117433485,32.9004022549204,30.));
#15168=CARTESIAN_POINT('Origin',(64.2032397694018,30.,30.));
#15169=CARTESIAN_POINT('',(64.2032397694018,34.,30.));
#15170=CARTESIAN_POINT('Origin',(35.8,34.,30.));
#15171=CARTESIAN_POINT('',(37.3967602305982,34.,30.));
#15172=CARTESIAN_POINT('Origin',(37.3967602305982,30.,30.));
#15173=CARTESIAN_POINT('',(34.6421882566514,32.9004022549204,30.));
#15174=CARTESIAN_POINT('Origin',(0.,0.,30.));
#15175=CARTESIAN_POINT('',(0.,0.,30.));
#15176=CARTESIAN_POINT('',(0.,0.,30.));
#15177=CARTESIAN_POINT('',(0.,0.,30.));
#15178=CARTESIAN_POINT('Origin',(2.06592898046005,-2.17530169119028,30.));
#15179=CARTESIAN_POINT('',(2.06592898046005,-2.17530169119028,30.));
#15180=CARTESIAN_POINT('',(2.06592898046005,-2.17530169119028,30.));
#15181=CARTESIAN_POINT('',(2.06592898046005,-2.17530169119028,30.));
#15182=CARTESIAN_POINT('Origin',(2.06592898046005,-2.17530169119028,30.));
#15183=CARTESIAN_POINT('',(36.7081172371115,30.7251005637301,30.));
#15184=CARTESIAN_POINT('',(2.06592898046005,-2.17530169119028,30.));
#15185=CARTESIAN_POINT('Origin',(37.3967602305982,30.,30.));
#15186=CARTESIAN_POINT('',(37.3967602305982,31.,30.));
#15187=CARTESIAN_POINT('Origin',(35.8,31.,30.));
#15188=CARTESIAN_POINT('',(64.2032397694018,31.,30.));
#15189=CARTESIAN_POINT('Origin',(64.2032397694018,30.,30.));
#15190=CARTESIAN_POINT('Origin',(64.2032397694018,30.,30.));
#15191=CARTESIAN_POINT('Origin',(64.2032397694018,30.,0.));
#17973=UNCERTAINTY_MEASURE_WITH_UNIT(LENGTH_MEASURE(0.01),#18007,
'DISTANCE_ACCURACY_VALUE',
'Maximum model space distance between geometric entities at asserted c
onnectivities');
#17986=UNCERTAINTY_MEASURE_WITH_UNIT(LENGTH_MEASURE(0.01),#18007,
'DISTANCE_ACCURACY_VALUE',
'Maximum model space distance between geometric entities at asserted c
onnectivities');
#17993=(
GEOMETRIC_REPRESENTATION_CONTEXT(3)
GLOBAL_UNCERTAINTY_ASSIGNED_CONTEXT((#17973))
GLOBAL_UNIT_ASSIGNED_CONTEXT((#18007,#18009,#18010))
REPRESENTATION_CONTEXT('','3D')
);
#18006=(
GEOMETRIC_REPRESENTATION_CONTEXT(3)
GLOBAL_UNCERTAINTY_ASSIGNED_CONTEXT((#17986))
GLOBAL_UNIT_ASSIGNED_CONTEXT((#18007,#18009,#18010))
REPRESENTATION_CONTEXT('','3D')
);
#18007=(
LENGTH_UNIT()
NAMED_UNIT(*)
SI_UNIT(.MILLI.,.METRE.)
);
#18009=(
NAMED_UNIT(*)
PLANE_ANGLE_UNIT()
SI_UNIT($,.RADIAN.)
);
#18010=(
NAMED_UNIT(*)
SI_UNIT($,.STERADIAN.)
SOLID_ANGLE_UNIT()
);
#18017=SHAPE_DEFINITION_REPRESENTATION(#18036,#18076);
#18036=PRODUCT_DEFINITION_SHAPE('',$,#18096);
#18076=SHAPE_REPRESENTATION('',(#10211),#17993);
#18089=PRODUCT_DEFINITION_CONTEXT('part definition',#18148,'design');
#18096=PRODUCT_DEFINITION('Catch Tray','Catch Tray',#18115,#18089);
#18115=PRODUCT_DEFINITION_FORMATION('',$,#18156);
#18148=APPLICATION_CONTEXT(
'Core Data for Automotive Mechanical Design Process');
#18149=PRODUCT_CONTEXT('part definition',#18148,'mechanical');
#18156=PRODUCT('Catch Tray','Catch Tray',$,(#18149));
#18170=PRESENTATION_STYLE_ASSIGNMENT((#18174));
#18174=SURFACE_STYLE_USAGE(.BOTH.,#18178);
#18178=SURFACE_SIDE_STYLE('',(#18182));
#18182=SURFACE_STYLE_FILL_AREA(#18186);
#18186=FILL_AREA_STYLE('Opaque(227,224,212)',(#18190));
#18190=FILL_AREA_STYLE_COLOUR('Opaque(227,224,212)',#18194);
#18194=COLOUR_RGB('Opaque(227,224,212)',0.890196078431372,0.87843137254902,
0.831372549019608);
ENDSEC;
END-ISO-10303-21;
